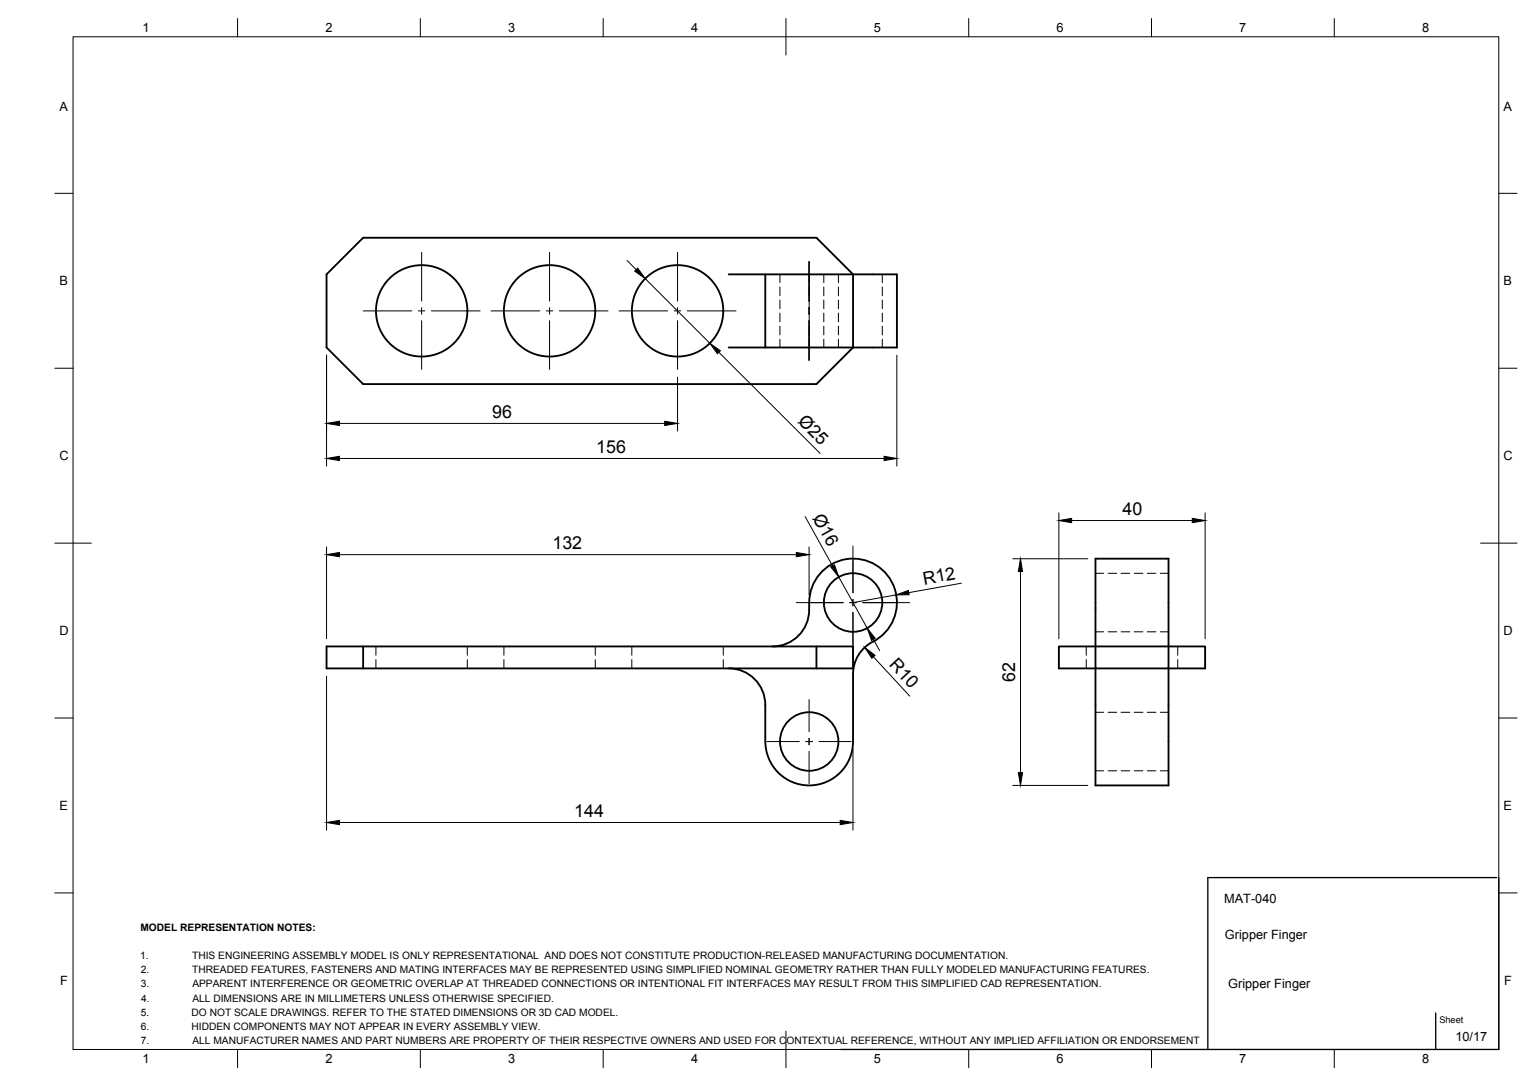
ISO-10303-21;
HEADER;
/* Generated by software containing ST-Developer
 * from STEP Tools, Inc. (www.steptools.com) 
 */

FILE_DESCRIPTION(
/* description */ ('STEP AP214'),
/* implementation_level */ '2;1');

FILE_NAME(
/* name */ 'Gripper Finger.step',
/* time_stamp */ '2026-11-14T21:53:28-08:00',
/* author */ (''),
/* organization */ (''),
/* preprocessor_version */ 'ST-DEVELOPER v20.2',
/* originating_system */ 'Autodesk Translation Framework v15.17.0.0',
/* authorisation */ '');

FILE_SCHEMA (('AUTOMOTIVE_DESIGN { 1 0 10303 214 3 1 1 }'));
ENDSEC;

DATA;
#10=MECHANICAL_DESIGN_GEOMETRIC_PRESENTATION_REPRESENTATION('',(#330),#20176);
#298=SHAPE_REPRESENTATION_RELATIONSHIP('SRR','None',#20261,#310);
#310=ADVANCED_BREP_SHAPE_REPRESENTATION('',(#357),#20167);
#330=STYLED_ITEM('',(#20337),#357);
#357=MANIFOLD_SOLID_BREP('Body1',#10948);
#536=FACE_BOUND('',#2109,.T.);
#537=FACE_BOUND('',#2110,.T.);
#538=FACE_BOUND('',#2111,.T.);
#539=FACE_BOUND('',#2117,.T.);
#540=FACE_BOUND('',#2118,.T.);
#541=FACE_BOUND('',#2119,.T.);
#542=FACE_BOUND('',#2125,.T.);
#543=FACE_BOUND('',#2126,.T.);
#544=FACE_BOUND('',#2128,.T.);
#545=FACE_BOUND('',#2129,.T.);
#826=PLANE('',#11930);
#827=PLANE('',#11931);
#828=PLANE('',#11932);
#829=PLANE('',#11933);
#830=PLANE('',#11934);
#831=PLANE('',#11935);
#832=PLANE('',#11936);
#833=PLANE('',#11940);
#834=PLANE('',#11941);
#835=PLANE('',#11942);
#836=PLANE('',#11946);
#837=PLANE('',#11951);
#838=PLANE('',#11952);
#839=PLANE('',#11953);
#1354=FACE_OUTER_BOUND('',#2102,.T.);
#1355=FACE_OUTER_BOUND('',#2103,.T.);
#1356=FACE_OUTER_BOUND('',#2104,.T.);
#1357=FACE_OUTER_BOUND('',#2105,.T.);
#1358=FACE_OUTER_BOUND('',#2106,.T.);
#1359=FACE_OUTER_BOUND('',#2107,.T.);
#1360=FACE_OUTER_BOUND('',#2108,.T.);
#1361=FACE_OUTER_BOUND('',#2112,.T.);
#1362=FACE_OUTER_BOUND('',#2113,.T.);
#1363=FACE_OUTER_BOUND('',#2114,.T.);
#1364=FACE_OUTER_BOUND('',#2115,.T.);
#1365=FACE_OUTER_BOUND('',#2116,.T.);
#1366=FACE_OUTER_BOUND('',#2120,.T.);
#1367=FACE_OUTER_BOUND('',#2121,.T.);
#1368=FACE_OUTER_BOUND('',#2122,.T.);
#1369=FACE_OUTER_BOUND('',#2123,.T.);
#1370=FACE_OUTER_BOUND('',#2124,.T.);
#1371=FACE_OUTER_BOUND('',#2127,.T.);
#1372=FACE_OUTER_BOUND('',#2130,.T.);
#1373=FACE_OUTER_BOUND('',#2131,.T.);
#1374=FACE_OUTER_BOUND('',#2132,.T.);
#1375=FACE_OUTER_BOUND('',#2133,.T.);
#1376=FACE_OUTER_BOUND('',#2134,.T.);
#1377=FACE_OUTER_BOUND('',#2135,.T.);
#2102=EDGE_LOOP('',(#9561,#9562,#9563,#9564));
#2103=EDGE_LOOP('',(#9565,#9566,#9567,#9568));
#2104=EDGE_LOOP('',(#9569,#9570,#9571,#9572));
#2105=EDGE_LOOP('',(#9573,#9574,#9575,#9576));
#2106=EDGE_LOOP('',(#9577,#9578,#9579,#9580));
#2107=EDGE_LOOP('',(#9581,#9582,#9583,#9584));
#2108=EDGE_LOOP('',(#9585,#9586,#9587,#9588,#9589,#9590,#9591,#9592,#9593,
#9594));
#2109=EDGE_LOOP('',(#9595));
#2110=EDGE_LOOP('',(#9596));
#2111=EDGE_LOOP('',(#9597));
#2112=EDGE_LOOP('',(#9598,#9599,#9600,#9601));
#2113=EDGE_LOOP('',(#9602,#9603,#9604,#9605));
#2114=EDGE_LOOP('',(#9606,#9607,#9608,#9609));
#2115=EDGE_LOOP('',(#9610,#9611,#9612,#9613));
#2116=EDGE_LOOP('',(#9614,#9615,#9616,#9617,#9618,#9619,#9620,#9621,#9622,
#9623));
#2117=EDGE_LOOP('',(#9624));
#2118=EDGE_LOOP('',(#9625));
#2119=EDGE_LOOP('',(#9626));
#2120=EDGE_LOOP('',(#9627,#9628,#9629,#9630));
#2121=EDGE_LOOP('',(#9631,#9632,#9633,#9634));
#2122=EDGE_LOOP('',(#9635,#9636,#9637,#9638));
#2123=EDGE_LOOP('',(#9639,#9640,#9641,#9642));
#2124=EDGE_LOOP('',(#9643,#9644,#9645,#9646,#9647,#9648,#9649,#9650,#9651,
#9652,#9653));
#2125=EDGE_LOOP('',(#9654));
#2126=EDGE_LOOP('',(#9655));
#2127=EDGE_LOOP('',(#9656,#9657,#9658,#9659,#9660,#9661,#9662,#9663,#9664,
#9665,#9666));
#2128=EDGE_LOOP('',(#9667));
#2129=EDGE_LOOP('',(#9668));
#2130=EDGE_LOOP('',(#9669,#9670,#9671,#9672));
#2131=EDGE_LOOP('',(#9673,#9674,#9675,#9676));
#2132=EDGE_LOOP('',(#9677,#9678,#9679,#9680));
#2133=EDGE_LOOP('',(#9681,#9682,#9683,#9684));
#2134=EDGE_LOOP('',(#9685,#9686,#9687,#9688));
#2135=EDGE_LOOP('',(#9689,#9690,#9691,#9692));
#3088=LINE('',#19463,#4076);
#3089=LINE('',#19469,#4077);
#3090=LINE('',#19475,#4078);
#3091=LINE('',#19482,#4079);
#3092=LINE('',#19485,#4080);
#3093=LINE('',#19490,#4081);
#3094=LINE('',#19496,#4082);
#3095=LINE('',#19501,#4083);
#3096=LINE('',#19503,#4084);
#3097=LINE('',#19505,#4085);
#3098=LINE('',#19507,#4086);
#3099=LINE('',#19509,#4087);
#3100=LINE('',#19511,#4088);
#3101=LINE('',#19513,#4089);
#3102=LINE('',#19515,#4090);
#3103=LINE('',#19517,#4091);
#3104=LINE('',#19518,#4092);
#3105=LINE('',#19521,#4093);
#3106=LINE('',#19523,#4094);
#3107=LINE('',#19524,#4095);
#3108=LINE('',#19527,#4096);
#3109=LINE('',#19529,#4097);
#3110=LINE('',#19530,#4098);
#3111=LINE('',#19534,#4099);
#3112=LINE('',#19536,#4100);
#3113=LINE('',#19538,#4101);
#3114=LINE('',#19539,#4102);
#3115=LINE('',#19542,#4103);
#3116=LINE('',#19544,#4104);
#3117=LINE('',#19545,#4105);
#3118=LINE('',#19548,#4106);
#3119=LINE('',#19550,#4107);
#3120=LINE('',#19552,#4108);
#3121=LINE('',#19554,#4109);
#3122=LINE('',#19555,#4110);
#3123=LINE('',#19556,#4111);
#3124=LINE('',#19557,#4112);
#3125=LINE('',#19561,#4113);
#3126=LINE('',#19563,#4114);
#3127=LINE('',#19565,#4115);
#3128=LINE('',#19566,#4116);
#3129=LINE('',#19575,#4117);
#3130=LINE('',#19577,#4118);
#3131=LINE('',#19581,#4119);
#3132=LINE('',#19584,#4120);
#3133=LINE('',#19590,#4121);
#4076=VECTOR('',#14642,12.5);
#4077=VECTOR('',#14649,12.5);
#4078=VECTOR('',#14656,12.5);
#4079=VECTOR('',#14663,1000.);
#4080=VECTOR('',#14666,1000.);
#4081=VECTOR('',#14671,8.);
#4082=VECTOR('',#14678,8.);
#4083=VECTOR('',#14683,1000.);
#4084=VECTOR('',#14684,1000.);
#4085=VECTOR('',#14685,1000.);
#4086=VECTOR('',#14686,1000.);
#4087=VECTOR('',#14687,1000.);
#4088=VECTOR('',#14688,1000.);
#4089=VECTOR('',#14689,1000.);
#4090=VECTOR('',#14690,1000.);
#4091=VECTOR('',#14691,1000.);
#4092=VECTOR('',#14692,1000.);
#4093=VECTOR('',#14695,1000.);
#4094=VECTOR('',#14696,1000.);
#4095=VECTOR('',#14697,1000.);
#4096=VECTOR('',#14700,1000.);
#4097=VECTOR('',#14701,1000.);
#4098=VECTOR('',#14702,1000.);
#4099=VECTOR('',#14705,1000.);
#4100=VECTOR('',#14706,1000.);
#4101=VECTOR('',#14707,1000.);
#4102=VECTOR('',#14708,1000.);
#4103=VECTOR('',#14711,1000.);
#4104=VECTOR('',#14712,1000.);
#4105=VECTOR('',#14713,1000.);
#4106=VECTOR('',#14716,1000.);
#4107=VECTOR('',#14717,1000.);
#4108=VECTOR('',#14718,1000.);
#4109=VECTOR('',#14719,1000.);
#4110=VECTOR('',#14720,1000.);
#4111=VECTOR('',#14721,1000.);
#4112=VECTOR('',#14722,1000.);
#4113=VECTOR('',#14725,1000.);
#4114=VECTOR('',#14726,1000.);
#4115=VECTOR('',#14727,1000.);
#4116=VECTOR('',#14728,1000.);
#4117=VECTOR('',#14743,1000.);
#4118=VECTOR('',#14746,1000.);
#4119=VECTOR('',#14751,1000.);
#4120=VECTOR('',#14756,1000.);
#4121=VECTOR('',#14767,1000.);
#4615=CIRCLE('',#11913,12.5);
#4616=CIRCLE('',#11914,12.5);
#4617=CIRCLE('',#11916,12.5);
#4618=CIRCLE('',#11917,12.5);
#4619=CIRCLE('',#11919,12.5);
#4620=CIRCLE('',#11920,12.5);
#4621=CIRCLE('',#11922,12.);
#4622=CIRCLE('',#11923,12.);
#4623=CIRCLE('',#11925,8.);
#4624=CIRCLE('',#11926,8.);
#4625=CIRCLE('',#11928,8.);
#4626=CIRCLE('',#11929,8.);
#4627=CIRCLE('',#11938,12.);
#4628=CIRCLE('',#11939,12.);
#4629=CIRCLE('',#11943,10.);
#4630=CIRCLE('',#11944,10.);
#4631=CIRCLE('',#11945,10.);
#4632=CIRCLE('',#11947,10.);
#4633=CIRCLE('',#11948,10.);
#4634=CIRCLE('',#11949,10.);
#5490=VERTEX_POINT('',#19460);
#5491=VERTEX_POINT('',#19462);
#5492=VERTEX_POINT('',#19466);
#5493=VERTEX_POINT('',#19468);
#5494=VERTEX_POINT('',#19472);
#5495=VERTEX_POINT('',#19474);
#5496=VERTEX_POINT('',#19478);
#5497=VERTEX_POINT('',#19479);
#5498=VERTEX_POINT('',#19481);
#5499=VERTEX_POINT('',#19483);
#5500=VERTEX_POINT('',#19487);
#5501=VERTEX_POINT('',#19489);
#5502=VERTEX_POINT('',#19493);
#5503=VERTEX_POINT('',#19495);
#5504=VERTEX_POINT('',#19499);
#5505=VERTEX_POINT('',#19500);
#5506=VERTEX_POINT('',#19502);
#5507=VERTEX_POINT('',#19504);
#5508=VERTEX_POINT('',#19506);
#5509=VERTEX_POINT('',#19508);
#5510=VERTEX_POINT('',#19510);
#5511=VERTEX_POINT('',#19512);
#5512=VERTEX_POINT('',#19514);
#5513=VERTEX_POINT('',#19516);
#5514=VERTEX_POINT('',#19520);
#5515=VERTEX_POINT('',#19522);
#5516=VERTEX_POINT('',#19526);
#5517=VERTEX_POINT('',#19528);
#5518=VERTEX_POINT('',#19532);
#5519=VERTEX_POINT('',#19533);
#5520=VERTEX_POINT('',#19535);
#5521=VERTEX_POINT('',#19537);
#5522=VERTEX_POINT('',#19541);
#5523=VERTEX_POINT('',#19543);
#5524=VERTEX_POINT('',#19547);
#5525=VERTEX_POINT('',#19549);
#5526=VERTEX_POINT('',#19551);
#5527=VERTEX_POINT('',#19553);
#5528=VERTEX_POINT('',#19559);
#5529=VERTEX_POINT('',#19560);
#5530=VERTEX_POINT('',#19562);
#5531=VERTEX_POINT('',#19564);
#5532=VERTEX_POINT('',#19574);
#5533=VERTEX_POINT('',#19580);
#6891=EDGE_CURVE('',#5490,#5490,#4615,.T.);
#6892=EDGE_CURVE('',#5490,#5491,#3088,.T.);
#6893=EDGE_CURVE('',#5491,#5491,#4616,.T.);
#6894=EDGE_CURVE('',#5492,#5492,#4617,.T.);
#6895=EDGE_CURVE('',#5492,#5493,#3089,.T.);
#6896=EDGE_CURVE('',#5493,#5493,#4618,.T.);
#6897=EDGE_CURVE('',#5494,#5494,#4619,.T.);
#6898=EDGE_CURVE('',#5494,#5495,#3090,.T.);
#6899=EDGE_CURVE('',#5495,#5495,#4620,.T.);
#6900=EDGE_CURVE('',#5496,#5497,#4621,.T.);
#6901=EDGE_CURVE('',#5497,#5498,#3091,.T.);
#6902=EDGE_CURVE('',#5498,#5499,#4622,.T.);
#6903=EDGE_CURVE('',#5499,#5496,#3092,.T.);
#6904=EDGE_CURVE('',#5500,#5500,#4623,.T.);
#6905=EDGE_CURVE('',#5500,#5501,#3093,.T.);
#6906=EDGE_CURVE('',#5501,#5501,#4624,.T.);
#6907=EDGE_CURVE('',#5502,#5502,#4625,.T.);
#6908=EDGE_CURVE('',#5502,#5503,#3094,.T.);
#6909=EDGE_CURVE('',#5503,#5503,#4626,.T.);
#6910=EDGE_CURVE('',#5504,#5505,#3095,.T.);
#6911=EDGE_CURVE('',#5505,#5506,#3096,.T.);
#6912=EDGE_CURVE('',#5507,#5506,#3097,.T.);
#6913=EDGE_CURVE('',#5508,#5507,#3098,.T.);
#6914=EDGE_CURVE('',#5508,#5509,#3099,.T.);
#6915=EDGE_CURVE('',#5509,#5510,#3100,.T.);
#6916=EDGE_CURVE('',#5511,#5510,#3101,.T.);
#6917=EDGE_CURVE('',#5511,#5512,#3102,.T.);
#6918=EDGE_CURVE('',#5513,#5512,#3103,.T.);
#6919=EDGE_CURVE('',#5504,#5513,#3104,.T.);
#6920=EDGE_CURVE('',#5513,#5514,#3105,.T.);
#6921=EDGE_CURVE('',#5512,#5515,#3106,.T.);
#6922=EDGE_CURVE('',#5515,#5514,#3107,.T.);
#6923=EDGE_CURVE('',#5508,#5516,#3108,.T.);
#6924=EDGE_CURVE('',#5517,#5516,#3109,.T.);
#6925=EDGE_CURVE('',#5517,#5509,#3110,.T.);
#6926=EDGE_CURVE('',#5518,#5519,#3111,.T.);
#6927=EDGE_CURVE('',#5518,#5520,#3112,.T.);
#6928=EDGE_CURVE('',#5521,#5520,#3113,.T.);
#6929=EDGE_CURVE('',#5521,#5519,#3114,.T.);
#6930=EDGE_CURVE('',#5510,#5522,#3115,.T.);
#6931=EDGE_CURVE('',#5523,#5522,#3116,.T.);
#6932=EDGE_CURVE('',#5523,#5511,#3117,.T.);
#6933=EDGE_CURVE('',#5524,#5516,#3118,.T.);
#6934=EDGE_CURVE('',#5524,#5525,#3119,.T.);
#6935=EDGE_CURVE('',#5525,#5526,#3120,.T.);
#6936=EDGE_CURVE('',#5527,#5526,#3121,.T.);
#6937=EDGE_CURVE('',#5514,#5527,#3122,.T.);
#6938=EDGE_CURVE('',#5515,#5523,#3123,.T.);
#6939=EDGE_CURVE('',#5522,#5517,#3124,.T.);
#6940=EDGE_CURVE('',#5528,#5529,#3125,.T.);
#6941=EDGE_CURVE('',#5528,#5530,#3126,.T.);
#6942=EDGE_CURVE('',#5531,#5530,#3127,.T.);
#6943=EDGE_CURVE('',#5529,#5531,#3128,.T.);
#6944=EDGE_CURVE('',#5519,#5531,#4627,.T.);
#6945=EDGE_CURVE('',#5529,#5521,#4628,.T.);
#6946=EDGE_CURVE('',#5520,#5499,#4629,.T.);
#6947=EDGE_CURVE('',#5532,#5498,#3129,.T.);
#6948=EDGE_CURVE('',#5532,#5505,#4630,.T.);
#6949=EDGE_CURVE('',#5504,#5527,#3130,.T.);
#6950=EDGE_CURVE('',#5526,#5528,#4631,.T.);
#6951=EDGE_CURVE('',#5497,#5533,#3131,.T.);
#6952=EDGE_CURVE('',#5496,#5518,#4632,.T.);
#6953=EDGE_CURVE('',#5530,#5525,#4633,.T.);
#6954=EDGE_CURVE('',#5507,#5524,#3132,.T.);
#6955=EDGE_CURVE('',#5506,#5533,#4634,.T.);
#6956=EDGE_CURVE('',#5533,#5532,#3133,.T.);
#9561=ORIENTED_EDGE('',*,*,#6891,.T.);
#9562=ORIENTED_EDGE('',*,*,#6892,.T.);
#9563=ORIENTED_EDGE('',*,*,#6893,.T.);
#9564=ORIENTED_EDGE('',*,*,#6892,.F.);
#9565=ORIENTED_EDGE('',*,*,#6894,.T.);
#9566=ORIENTED_EDGE('',*,*,#6895,.T.);
#9567=ORIENTED_EDGE('',*,*,#6896,.T.);
#9568=ORIENTED_EDGE('',*,*,#6895,.F.);
#9569=ORIENTED_EDGE('',*,*,#6897,.T.);
#9570=ORIENTED_EDGE('',*,*,#6898,.T.);
#9571=ORIENTED_EDGE('',*,*,#6899,.T.);
#9572=ORIENTED_EDGE('',*,*,#6898,.F.);
#9573=ORIENTED_EDGE('',*,*,#6900,.T.);
#9574=ORIENTED_EDGE('',*,*,#6901,.T.);
#9575=ORIENTED_EDGE('',*,*,#6902,.T.);
#9576=ORIENTED_EDGE('',*,*,#6903,.T.);
#9577=ORIENTED_EDGE('',*,*,#6904,.F.);
#9578=ORIENTED_EDGE('',*,*,#6905,.T.);
#9579=ORIENTED_EDGE('',*,*,#6906,.F.);
#9580=ORIENTED_EDGE('',*,*,#6905,.F.);
#9581=ORIENTED_EDGE('',*,*,#6907,.T.);
#9582=ORIENTED_EDGE('',*,*,#6908,.T.);
#9583=ORIENTED_EDGE('',*,*,#6909,.T.);
#9584=ORIENTED_EDGE('',*,*,#6908,.F.);
#9585=ORIENTED_EDGE('',*,*,#6910,.T.);
#9586=ORIENTED_EDGE('',*,*,#6911,.T.);
#9587=ORIENTED_EDGE('',*,*,#6912,.F.);
#9588=ORIENTED_EDGE('',*,*,#6913,.F.);
#9589=ORIENTED_EDGE('',*,*,#6914,.T.);
#9590=ORIENTED_EDGE('',*,*,#6915,.T.);
#9591=ORIENTED_EDGE('',*,*,#6916,.F.);
#9592=ORIENTED_EDGE('',*,*,#6917,.T.);
#9593=ORIENTED_EDGE('',*,*,#6918,.F.);
#9594=ORIENTED_EDGE('',*,*,#6919,.F.);
#9595=ORIENTED_EDGE('',*,*,#6893,.F.);
#9596=ORIENTED_EDGE('',*,*,#6896,.F.);
#9597=ORIENTED_EDGE('',*,*,#6899,.F.);
#9598=ORIENTED_EDGE('',*,*,#6920,.F.);
#9599=ORIENTED_EDGE('',*,*,#6918,.T.);
#9600=ORIENTED_EDGE('',*,*,#6921,.T.);
#9601=ORIENTED_EDGE('',*,*,#6922,.T.);
#9602=ORIENTED_EDGE('',*,*,#6914,.F.);
#9603=ORIENTED_EDGE('',*,*,#6923,.T.);
#9604=ORIENTED_EDGE('',*,*,#6924,.F.);
#9605=ORIENTED_EDGE('',*,*,#6925,.T.);
#9606=ORIENTED_EDGE('',*,*,#6926,.F.);
#9607=ORIENTED_EDGE('',*,*,#6927,.T.);
#9608=ORIENTED_EDGE('',*,*,#6928,.F.);
#9609=ORIENTED_EDGE('',*,*,#6929,.T.);
#9610=ORIENTED_EDGE('',*,*,#6916,.T.);
#9611=ORIENTED_EDGE('',*,*,#6930,.T.);
#9612=ORIENTED_EDGE('',*,*,#6931,.F.);
#9613=ORIENTED_EDGE('',*,*,#6932,.T.);
#9614=ORIENTED_EDGE('',*,*,#6924,.T.);
#9615=ORIENTED_EDGE('',*,*,#6933,.F.);
#9616=ORIENTED_EDGE('',*,*,#6934,.T.);
#9617=ORIENTED_EDGE('',*,*,#6935,.T.);
#9618=ORIENTED_EDGE('',*,*,#6936,.F.);
#9619=ORIENTED_EDGE('',*,*,#6937,.F.);
#9620=ORIENTED_EDGE('',*,*,#6922,.F.);
#9621=ORIENTED_EDGE('',*,*,#6938,.T.);
#9622=ORIENTED_EDGE('',*,*,#6931,.T.);
#9623=ORIENTED_EDGE('',*,*,#6939,.T.);
#9624=ORIENTED_EDGE('',*,*,#6891,.F.);
#9625=ORIENTED_EDGE('',*,*,#6894,.F.);
#9626=ORIENTED_EDGE('',*,*,#6897,.F.);
#9627=ORIENTED_EDGE('',*,*,#6940,.F.);
#9628=ORIENTED_EDGE('',*,*,#6941,.T.);
#9629=ORIENTED_EDGE('',*,*,#6942,.F.);
#9630=ORIENTED_EDGE('',*,*,#6943,.F.);
#9631=ORIENTED_EDGE('',*,*,#6943,.T.);
#9632=ORIENTED_EDGE('',*,*,#6944,.F.);
#9633=ORIENTED_EDGE('',*,*,#6929,.F.);
#9634=ORIENTED_EDGE('',*,*,#6945,.F.);
#9635=ORIENTED_EDGE('',*,*,#6915,.F.);
#9636=ORIENTED_EDGE('',*,*,#6925,.F.);
#9637=ORIENTED_EDGE('',*,*,#6939,.F.);
#9638=ORIENTED_EDGE('',*,*,#6930,.F.);
#9639=ORIENTED_EDGE('',*,*,#6917,.F.);
#9640=ORIENTED_EDGE('',*,*,#6932,.F.);
#9641=ORIENTED_EDGE('',*,*,#6938,.F.);
#9642=ORIENTED_EDGE('',*,*,#6921,.F.);
#9643=ORIENTED_EDGE('',*,*,#6928,.T.);
#9644=ORIENTED_EDGE('',*,*,#6946,.T.);
#9645=ORIENTED_EDGE('',*,*,#6902,.F.);
#9646=ORIENTED_EDGE('',*,*,#6947,.F.);
#9647=ORIENTED_EDGE('',*,*,#6948,.T.);
#9648=ORIENTED_EDGE('',*,*,#6910,.F.);
#9649=ORIENTED_EDGE('',*,*,#6949,.T.);
#9650=ORIENTED_EDGE('',*,*,#6936,.T.);
#9651=ORIENTED_EDGE('',*,*,#6950,.T.);
#9652=ORIENTED_EDGE('',*,*,#6940,.T.);
#9653=ORIENTED_EDGE('',*,*,#6945,.T.);
#9654=ORIENTED_EDGE('',*,*,#6906,.T.);
#9655=ORIENTED_EDGE('',*,*,#6907,.F.);
#9656=ORIENTED_EDGE('',*,*,#6951,.F.);
#9657=ORIENTED_EDGE('',*,*,#6900,.F.);
#9658=ORIENTED_EDGE('',*,*,#6952,.T.);
#9659=ORIENTED_EDGE('',*,*,#6926,.T.);
#9660=ORIENTED_EDGE('',*,*,#6944,.T.);
#9661=ORIENTED_EDGE('',*,*,#6942,.T.);
#9662=ORIENTED_EDGE('',*,*,#6953,.T.);
#9663=ORIENTED_EDGE('',*,*,#6934,.F.);
#9664=ORIENTED_EDGE('',*,*,#6954,.F.);
#9665=ORIENTED_EDGE('',*,*,#6912,.T.);
#9666=ORIENTED_EDGE('',*,*,#6955,.T.);
#9667=ORIENTED_EDGE('',*,*,#6904,.T.);
#9668=ORIENTED_EDGE('',*,*,#6909,.F.);
#9669=ORIENTED_EDGE('',*,*,#6950,.F.);
#9670=ORIENTED_EDGE('',*,*,#6935,.F.);
#9671=ORIENTED_EDGE('',*,*,#6953,.F.);
#9672=ORIENTED_EDGE('',*,*,#6941,.F.);
#9673=ORIENTED_EDGE('',*,*,#6919,.T.);
#9674=ORIENTED_EDGE('',*,*,#6920,.T.);
#9675=ORIENTED_EDGE('',*,*,#6937,.T.);
#9676=ORIENTED_EDGE('',*,*,#6949,.F.);
#9677=ORIENTED_EDGE('',*,*,#6913,.T.);
#9678=ORIENTED_EDGE('',*,*,#6954,.T.);
#9679=ORIENTED_EDGE('',*,*,#6933,.T.);
#9680=ORIENTED_EDGE('',*,*,#6923,.F.);
#9681=ORIENTED_EDGE('',*,*,#6951,.T.);
#9682=ORIENTED_EDGE('',*,*,#6956,.T.);
#9683=ORIENTED_EDGE('',*,*,#6947,.T.);
#9684=ORIENTED_EDGE('',*,*,#6901,.F.);
#9685=ORIENTED_EDGE('',*,*,#6955,.F.);
#9686=ORIENTED_EDGE('',*,*,#6911,.F.);
#9687=ORIENTED_EDGE('',*,*,#6948,.F.);
#9688=ORIENTED_EDGE('',*,*,#6956,.F.);
#9689=ORIENTED_EDGE('',*,*,#6946,.F.);
#9690=ORIENTED_EDGE('',*,*,#6927,.F.);
#9691=ORIENTED_EDGE('',*,*,#6952,.F.);
#9692=ORIENTED_EDGE('',*,*,#6903,.F.);
#10311=CYLINDRICAL_SURFACE('',#11912,12.5);
#10312=CYLINDRICAL_SURFACE('',#11915,12.5);
#10313=CYLINDRICAL_SURFACE('',#11918,12.5);
#10314=CYLINDRICAL_SURFACE('',#11921,12.);
#10315=CYLINDRICAL_SURFACE('',#11924,8.);
#10316=CYLINDRICAL_SURFACE('',#11927,8.);
#10317=CYLINDRICAL_SURFACE('',#11937,12.);
#10318=CYLINDRICAL_SURFACE('',#11950,10.);
#10319=CYLINDRICAL_SURFACE('',#11954,10.);
#10320=CYLINDRICAL_SURFACE('',#11955,10.);
#10806=ADVANCED_FACE('',(#1354),#10311,.F.);
#10807=ADVANCED_FACE('',(#1355),#10312,.F.);
#10808=ADVANCED_FACE('',(#1356),#10313,.F.);
#10809=ADVANCED_FACE('',(#1357),#10314,.T.);
#10810=ADVANCED_FACE('',(#1358),#10315,.F.);
#10811=ADVANCED_FACE('',(#1359),#10316,.F.);
#10812=ADVANCED_FACE('',(#1360,#536,#537,#538),#826,.F.);
#10813=ADVANCED_FACE('',(#1361),#827,.T.);
#10814=ADVANCED_FACE('',(#1362),#828,.F.);
#10815=ADVANCED_FACE('',(#1363),#829,.F.);
#10816=ADVANCED_FACE('',(#1364),#830,.F.);
#10817=ADVANCED_FACE('',(#1365,#539,#540,#541),#831,.F.);
#10818=ADVANCED_FACE('',(#1366),#832,.F.);
#10819=ADVANCED_FACE('',(#1367),#10317,.T.);
#10820=ADVANCED_FACE('',(#1368),#833,.F.);
#10821=ADVANCED_FACE('',(#1369),#834,.T.);
#10822=ADVANCED_FACE('',(#1370,#542,#543),#835,.F.);
#10823=ADVANCED_FACE('',(#1371,#544,#545),#836,.F.);
#10824=ADVANCED_FACE('',(#1372),#10318,.F.);
#10825=ADVANCED_FACE('',(#1373),#837,.F.);
#10826=ADVANCED_FACE('',(#1374),#838,.F.);
#10827=ADVANCED_FACE('',(#1375),#839,.F.);
#10828=ADVANCED_FACE('',(#1376),#10319,.F.);
#10829=ADVANCED_FACE('',(#1377),#10320,.F.);
#10948=CLOSED_SHELL('',(#10806,#10807,#10808,#10809,#10810,#10811,#10812,
#10813,#10814,#10815,#10816,#10817,#10818,#10819,#10820,#10821,#10822,#10823,
#10824,#10825,#10826,#10827,#10828,#10829));
#11911=AXIS2_PLACEMENT_3D('',#19458,#14636,#14637);
#11912=AXIS2_PLACEMENT_3D('',#19459,#14638,#14639);
#11913=AXIS2_PLACEMENT_3D('',#19461,#14640,#14641);
#11914=AXIS2_PLACEMENT_3D('',#19464,#14643,#14644);
#11915=AXIS2_PLACEMENT_3D('',#19465,#14645,#14646);
#11916=AXIS2_PLACEMENT_3D('',#19467,#14647,#14648);
#11917=AXIS2_PLACEMENT_3D('',#19470,#14650,#14651);
#11918=AXIS2_PLACEMENT_3D('',#19471,#14652,#14653);
#11919=AXIS2_PLACEMENT_3D('',#19473,#14654,#14655);
#11920=AXIS2_PLACEMENT_3D('',#19476,#14657,#14658);
#11921=AXIS2_PLACEMENT_3D('',#19477,#14659,#14660);
#11922=AXIS2_PLACEMENT_3D('',#19480,#14661,#14662);
#11923=AXIS2_PLACEMENT_3D('',#19484,#14664,#14665);
#11924=AXIS2_PLACEMENT_3D('',#19486,#14667,#14668);
#11925=AXIS2_PLACEMENT_3D('',#19488,#14669,#14670);
#11926=AXIS2_PLACEMENT_3D('',#19491,#14672,#14673);
#11927=AXIS2_PLACEMENT_3D('',#19492,#14674,#14675);
#11928=AXIS2_PLACEMENT_3D('',#19494,#14676,#14677);
#11929=AXIS2_PLACEMENT_3D('',#19497,#14679,#14680);
#11930=AXIS2_PLACEMENT_3D('',#19498,#14681,#14682);
#11931=AXIS2_PLACEMENT_3D('',#19519,#14693,#14694);
#11932=AXIS2_PLACEMENT_3D('',#19525,#14698,#14699);
#11933=AXIS2_PLACEMENT_3D('',#19531,#14703,#14704);
#11934=AXIS2_PLACEMENT_3D('',#19540,#14709,#14710);
#11935=AXIS2_PLACEMENT_3D('',#19546,#14714,#14715);
#11936=AXIS2_PLACEMENT_3D('',#19558,#14723,#14724);
#11937=AXIS2_PLACEMENT_3D('',#19567,#14729,#14730);
#11938=AXIS2_PLACEMENT_3D('',#19568,#14731,#14732);
#11939=AXIS2_PLACEMENT_3D('',#19569,#14733,#14734);
#11940=AXIS2_PLACEMENT_3D('',#19570,#14735,#14736);
#11941=AXIS2_PLACEMENT_3D('',#19571,#14737,#14738);
#11942=AXIS2_PLACEMENT_3D('',#19572,#14739,#14740);
#11943=AXIS2_PLACEMENT_3D('',#19573,#14741,#14742);
#11944=AXIS2_PLACEMENT_3D('',#19576,#14744,#14745);
#11945=AXIS2_PLACEMENT_3D('',#19578,#14747,#14748);
#11946=AXIS2_PLACEMENT_3D('',#19579,#14749,#14750);
#11947=AXIS2_PLACEMENT_3D('',#19582,#14752,#14753);
#11948=AXIS2_PLACEMENT_3D('',#19583,#14754,#14755);
#11949=AXIS2_PLACEMENT_3D('',#19585,#14757,#14758);
#11950=AXIS2_PLACEMENT_3D('',#19586,#14759,#14760);
#11951=AXIS2_PLACEMENT_3D('',#19587,#14761,#14762);
#11952=AXIS2_PLACEMENT_3D('',#19588,#14763,#14764);
#11953=AXIS2_PLACEMENT_3D('',#19589,#14765,#14766);
#11954=AXIS2_PLACEMENT_3D('',#19591,#14768,#14769);
#11955=AXIS2_PLACEMENT_3D('',#19592,#14770,#14771);
#14636=DIRECTION('axis',(0.,0.,1.));
#14637=DIRECTION('refdir',(1.,0.,0.));
#14638=DIRECTION('center_axis',(1.,0.,0.));
#14639=DIRECTION('ref_axis',(0.,0.,-1.));
#14640=DIRECTION('center_axis',(-1.,0.,0.));
#14641=DIRECTION('ref_axis',(0.,0.,-1.));
#14642=DIRECTION('',(1.,0.,0.));
#14643=DIRECTION('center_axis',(1.,0.,0.));
#14644=DIRECTION('ref_axis',(0.,0.,1.));
#14645=DIRECTION('center_axis',(1.,0.,0.));
#14646=DIRECTION('ref_axis',(0.,0.,-1.));
#14647=DIRECTION('center_axis',(-1.,0.,0.));
#14648=DIRECTION('ref_axis',(0.,0.,-1.));
#14649=DIRECTION('',(1.,0.,0.));
#14650=DIRECTION('center_axis',(1.,0.,0.));
#14651=DIRECTION('ref_axis',(0.,0.,-1.));
#14652=DIRECTION('center_axis',(1.,0.,0.));
#14653=DIRECTION('ref_axis',(0.,0.,-1.));
#14654=DIRECTION('center_axis',(-1.,0.,0.));
#14655=DIRECTION('ref_axis',(0.,0.,-1.));
#14656=DIRECTION('',(1.,0.,0.));
#14657=DIRECTION('center_axis',(1.,0.,0.));
#14658=DIRECTION('ref_axis',(0.,0.,-1.));
#14659=DIRECTION('center_axis',(0.,1.,0.));
#14660=DIRECTION('ref_axis',(0.,0.,1.));
#14661=DIRECTION('center_axis',(3.46944695195361E-16,1.,0.));
#14662=DIRECTION('ref_axis',(-1.,3.46944695195361E-16,0.));
#14663=DIRECTION('',(-1.73472347597681E-16,1.,0.));
#14664=DIRECTION('center_axis',(1.73472347597681E-16,-1.,0.));
#14665=DIRECTION('ref_axis',(1.,1.73472347597681E-16,0.));
#14666=DIRECTION('',(0.,-1.,0.));
#14667=DIRECTION('center_axis',(0.,1.,0.));
#14668=DIRECTION('ref_axis',(0.,0.,1.));
#14669=DIRECTION('center_axis',(3.46944695195361E-16,1.,0.));
#14670=DIRECTION('ref_axis',(-1.,3.46944695195361E-16,0.));
#14671=DIRECTION('',(0.,1.,0.));
#14672=DIRECTION('center_axis',(1.73472347597681E-16,-1.,0.));
#14673=DIRECTION('ref_axis',(1.,1.73472347597681E-16,0.));
#14674=DIRECTION('center_axis',(0.,-1.,0.));
#14675=DIRECTION('ref_axis',(0.,0.,-1.));
#14676=DIRECTION('center_axis',(0.,1.,0.));
#14677=DIRECTION('ref_axis',(0.,0.,-1.));
#14678=DIRECTION('',(0.,-1.,0.));
#14679=DIRECTION('center_axis',(0.,-1.,0.));
#14680=DIRECTION('ref_axis',(0.,0.,1.));
#14681=DIRECTION('center_axis',(-1.,0.,0.));
#14682=DIRECTION('ref_axis',(0.,0.,1.));
#14683=DIRECTION('',(0.,0.,-1.));
#14684=DIRECTION('',(0.,-1.,5.01544256350842E-32));
#14685=DIRECTION('',(0.,0.,-1.));
#14686=DIRECTION('',(0.,0.707106781186548,0.707106781186548));
#14687=DIRECTION('',(0.,0.,-1.));
#14688=DIRECTION('',(0.,0.707106781186546,-0.707106781186549));
#14689=DIRECTION('',(0.,-1.,0.));
#14690=DIRECTION('',(0.,0.707106781186547,0.707106781186547));
#14691=DIRECTION('',(0.,0.,-1.));
#14692=DIRECTION('',(0.,0.707106781186547,-0.707106781186548));
#14693=DIRECTION('center_axis',(0.,1.,0.));
#14694=DIRECTION('ref_axis',(0.,0.,1.));
#14695=DIRECTION('',(-1.,0.,0.));
#14696=DIRECTION('',(-1.,0.,0.));
#14697=DIRECTION('',(0.,0.,1.));
#14698=DIRECTION('center_axis',(0.,1.,0.));
#14699=DIRECTION('ref_axis',(0.,0.,1.));
#14700=DIRECTION('',(-1.,0.,0.));
#14701=DIRECTION('',(0.,0.,1.));
#14702=DIRECTION('',(1.,0.,0.));
#14703=DIRECTION('center_axis',(-4.00320802148494E-16,0.,-1.));
#14704=DIRECTION('ref_axis',(-1.,0.,4.00320802148494E-16));
#14705=DIRECTION('',(-1.,0.,4.00320802148494E-16));
#14706=DIRECTION('',(0.,1.,0.));
#14707=DIRECTION('',(1.,0.,-4.00320802148494E-16));
#14708=DIRECTION('',(0.,-1.,0.));
#14709=DIRECTION('center_axis',(0.,0.,1.));
#14710=DIRECTION('ref_axis',(1.,0.,0.));
#14711=DIRECTION('',(-1.,0.,0.));
#14712=DIRECTION('',(0.,-1.,0.));
#14713=DIRECTION('',(1.,0.,0.));
#14714=DIRECTION('center_axis',(1.,0.,0.));
#14715=DIRECTION('ref_axis',(0.,0.,-1.));
#14716=DIRECTION('',(0.,-0.707106781186548,-0.707106781186548));
#14717=DIRECTION('',(0.,0.,-1.));
#14718=DIRECTION('',(0.,1.,0.));
#14719=DIRECTION('',(0.,0.,-1.));
#14720=DIRECTION('',(0.,-0.707106781186547,0.707106781186548));
#14721=DIRECTION('',(0.,-0.707106781186547,-0.707106781186547));
#14722=DIRECTION('',(0.,-0.707106781186546,0.707106781186549));
#14723=DIRECTION('center_axis',(0.,0.,1.));
#14724=DIRECTION('ref_axis',(1.,0.,0.));
#14725=DIRECTION('',(-1.,0.,0.));
#14726=DIRECTION('',(0.,-1.,0.));
#14727=DIRECTION('',(1.,0.,0.));
#14728=DIRECTION('',(0.,-1.,0.));
#14729=DIRECTION('center_axis',(0.,-1.,0.));
#14730=DIRECTION('ref_axis',(0.,0.,-1.));
#14731=DIRECTION('center_axis',(0.,-1.,0.));
#14732=DIRECTION('ref_axis',(0.,0.,1.));
#14733=DIRECTION('center_axis',(0.,1.,0.));
#14734=DIRECTION('ref_axis',(0.,0.,-1.));
#14735=DIRECTION('center_axis',(0.,0.707106781186549,0.707106781186546));
#14736=DIRECTION('ref_axis',(-1.,0.,0.));
#14737=DIRECTION('center_axis',(0.,0.707106781186548,-0.707106781186548));
#14738=DIRECTION('ref_axis',(1.,0.,0.));
#14739=DIRECTION('center_axis',(0.,-1.,0.));
#14740=DIRECTION('ref_axis',(0.,0.,-1.));
#14741=DIRECTION('center_axis',(1.73472347597681E-16,-1.,0.));
#14742=DIRECTION('ref_axis',(1.,1.73472347597681E-16,0.));
#14743=DIRECTION('',(1.,2.89120579329468E-16,-2.89120579329468E-16));
#14744=DIRECTION('center_axis',(1.73472347597681E-16,-1.,0.));
#14745=DIRECTION('ref_axis',(1.,1.73472347597681E-16,0.));
#14746=DIRECTION('',(-1.,-1.73472347597681E-16,1.73472347597681E-16));
#14747=DIRECTION('center_axis',(0.,-1.,0.));
#14748=DIRECTION('ref_axis',(0.,0.,-1.));
#14749=DIRECTION('center_axis',(3.46944695195361E-16,1.,0.));
#14750=DIRECTION('ref_axis',(-1.,3.46944695195361E-16,0.));
#14751=DIRECTION('',(-1.,3.46944695195361E-16,2.89120579329468E-16));
#14752=DIRECTION('center_axis',(0.,1.,0.));
#14753=DIRECTION('ref_axis',(0.,0.,1.));
#14754=DIRECTION('center_axis',(0.,1.,0.));
#14755=DIRECTION('ref_axis',(0.,0.,1.));
#14756=DIRECTION('',(-1.,3.46944695195361E-16,3.46944695195361E-16));
#14757=DIRECTION('center_axis',(3.46944695195361E-16,1.,0.));
#14758=DIRECTION('ref_axis',(-1.,3.46944695195361E-16,0.));
#14759=DIRECTION('center_axis',(0.,1.,0.));
#14760=DIRECTION('ref_axis',(0.,0.,1.));
#14761=DIRECTION('center_axis',(0.,-0.707106781186548,-0.707106781186547));
#14762=DIRECTION('ref_axis',(0.,0.707106781186547,-0.707106781186548));
#14763=DIRECTION('center_axis',(0.,0.707106781186547,-0.707106781186548));
#14764=DIRECTION('ref_axis',(0.,0.707106781186548,0.707106781186547));
#14765=DIRECTION('center_axis',(2.89120579329468E-16,5.01544256350842E-32,
1.));
#14766=DIRECTION('ref_axis',(1.,-1.72766579818696E-64,-2.89120579329468E-16));
#14767=DIRECTION('',(0.,1.,-5.01544256350842E-32));
#14768=DIRECTION('center_axis',(0.,-1.,5.01544256350842E-32));
#14769=DIRECTION('ref_axis',(0.,-5.01544256350842E-32,-1.));
#14770=DIRECTION('center_axis',(0.,1.,0.));
#14771=DIRECTION('ref_axis',(0.,0.,1.));
#19458=CARTESIAN_POINT('',(0.,0.,0.));
#19459=CARTESIAN_POINT('Origin',(-38.001,20.,-48.));
#19460=CARTESIAN_POINT('',(-6.,20.,-35.5));
#19461=CARTESIAN_POINT('Origin',(-6.,20.,-48.));
#19462=CARTESIAN_POINT('',(0.,20.,-35.5));
#19463=CARTESIAN_POINT('',(-38.001,20.,-35.5));
#19464=CARTESIAN_POINT('Origin',(0.,20.,-48.));
#19465=CARTESIAN_POINT('Origin',(-38.001,20.,-118.));
#19466=CARTESIAN_POINT('',(-6.,20.,-105.5));
#19467=CARTESIAN_POINT('Origin',(-6.,20.,-118.));
#19468=CARTESIAN_POINT('',(0.,20.,-105.5));
#19469=CARTESIAN_POINT('',(-38.001,20.,-105.5));
#19470=CARTESIAN_POINT('Origin',(0.,20.,-118.));
#19471=CARTESIAN_POINT('Origin',(-38.001,20.,-83.));
#19472=CARTESIAN_POINT('',(-6.,20.,-70.5));
#19473=CARTESIAN_POINT('Origin',(-6.,20.,-83.));
#19474=CARTESIAN_POINT('',(0.,20.,-70.5));
#19475=CARTESIAN_POINT('',(-38.001,20.,-70.5));
#19476=CARTESIAN_POINT('Origin',(0.,20.,-83.));
#19477=CARTESIAN_POINT('Origin',(12.,-6.93889390390723E-15,3.46944695195361E-15));
#19478=CARTESIAN_POINT('',(1.31131748603704,10.,5.45454545454546));
#19479=CARTESIAN_POINT('',(12.,10.,-12.));
#19480=CARTESIAN_POINT('Origin',(12.,10.,3.46944695195361E-15));
#19481=CARTESIAN_POINT('',(12.,30.,-12.));
#19482=CARTESIAN_POINT('',(12.,-0.00100000000000794,-12.));
#19483=CARTESIAN_POINT('',(1.31131748603704,30.,5.45454545454546));
#19484=CARTESIAN_POINT('Origin',(12.,30.,3.46944695195361E-15));
#19485=CARTESIAN_POINT('',(1.31131748603704,-6.93889390390723E-15,5.45454545454546));
#19486=CARTESIAN_POINT('Origin',(12.,-6.93889390390723E-15,3.46944695195361E-15));
#19487=CARTESIAN_POINT('',(12.,10.,-8.));
#19488=CARTESIAN_POINT('Origin',(12.,10.,3.46944695195361E-15));
#19489=CARTESIAN_POINT('',(12.,30.,-8.));
#19490=CARTESIAN_POINT('',(12.,-6.93889390390723E-15,-8.));
#19491=CARTESIAN_POINT('Origin',(12.,30.,3.46944695195361E-15));
#19492=CARTESIAN_POINT('Origin',(-26.,40.,-12.));
#19493=CARTESIAN_POINT('',(-26.,30.,-4.));
#19494=CARTESIAN_POINT('Origin',(-26.,30.,-12.));
#19495=CARTESIAN_POINT('',(-26.,10.,-4.));
#19496=CARTESIAN_POINT('',(-26.,40.,-4.));
#19497=CARTESIAN_POINT('Origin',(-26.,10.,-12.));
#19498=CARTESIAN_POINT('Origin',(0.,40.,0.));
#19499=CARTESIAN_POINT('',(0.,30.,1.73472347597681E-15));
#19500=CARTESIAN_POINT('',(0.,30.,-22.));
#19501=CARTESIAN_POINT('',(-1.24683249835833E-15,30.,12.001));
#19502=CARTESIAN_POINT('',(4.87890977618477E-16,10.,-22.));
#19503=CARTESIAN_POINT('',(0.,10.,-22.));
#19504=CARTESIAN_POINT('',(3.46944695195361E-15,10.,1.73472347597681E-15));
#19505=CARTESIAN_POINT('',(4.87890977618477E-16,10.,12.001));
#19506=CARTESIAN_POINT('',(0.,0.,-10.));
#19507=CARTESIAN_POINT('',(0.,-1.22464679914735E-15,-10.));
#19508=CARTESIAN_POINT('',(0.,-6.93889390390723E-15,-134.));
#19509=CARTESIAN_POINT('',(0.,0.,0.));
#19510=CARTESIAN_POINT('',(0.,10.,-144.));
#19511=CARTESIAN_POINT('',(0.,10.,-144.));
#19512=CARTESIAN_POINT('',(0.,30.,-144.));
#19513=CARTESIAN_POINT('',(0.,40.,-144.));
#19514=CARTESIAN_POINT('',(0.,40.,-134.));
#19515=CARTESIAN_POINT('',(0.,40.,-134.));
#19516=CARTESIAN_POINT('',(0.,40.,-10.));
#19517=CARTESIAN_POINT('',(0.,40.,0.));
#19518=CARTESIAN_POINT('',(0.,30.,1.73472347597681E-15));
#19519=CARTESIAN_POINT('Origin',(-26.,40.,-12.));
#19520=CARTESIAN_POINT('',(-6.,40.,-10.));
#19521=CARTESIAN_POINT('',(24.001,40.,-10.));
#19522=CARTESIAN_POINT('',(-6.,40.,-134.));
#19523=CARTESIAN_POINT('',(-6.,40.,-134.));
#19524=CARTESIAN_POINT('',(-6.,40.,-24.));
#19525=CARTESIAN_POINT('Origin',(-26.,0.,-12.));
#19526=CARTESIAN_POINT('',(-6.,-1.22464679914735E-15,-10.));
#19527=CARTESIAN_POINT('',(24.001,-1.22464679914735E-15,-10.));
#19528=CARTESIAN_POINT('',(-6.,0.,-134.));
#19529=CARTESIAN_POINT('',(-6.,0.,-24.));
#19530=CARTESIAN_POINT('',(-26.,0.,-134.));
#19531=CARTESIAN_POINT('Origin',(0.,40.,0.));
#19532=CARTESIAN_POINT('',(-7.59591794226543,10.,2.37360262678768E-15));
#19533=CARTESIAN_POINT('',(-26.,10.,8.67361737988404E-15));
#19534=CARTESIAN_POINT('',(-6.,10.,1.73472347597681E-15));
#19535=CARTESIAN_POINT('',(-7.59591794226543,30.,3.27314145353471E-15));
#19536=CARTESIAN_POINT('',(-7.59591794226543,40.,3.04080396370184E-15));
#19537=CARTESIAN_POINT('',(-26.,30.,8.67361737988404E-15));
#19538=CARTESIAN_POINT('',(-6.,30.,1.73472347597681E-15));
#19539=CARTESIAN_POINT('',(-26.,40.,8.67361737988404E-15));
#19540=CARTESIAN_POINT('Origin',(0.,40.,-144.));
#19541=CARTESIAN_POINT('',(-6.,10.,-144.));
#19542=CARTESIAN_POINT('',(0.,10.,-144.));
#19543=CARTESIAN_POINT('',(-6.,30.,-144.));
#19544=CARTESIAN_POINT('',(-6.,40.,-144.));
#19545=CARTESIAN_POINT('',(0.,30.,-144.));
#19546=CARTESIAN_POINT('Origin',(-6.,40.,-24.));
#19547=CARTESIAN_POINT('',(-6.,10.,1.73472347597681E-15));
#19548=CARTESIAN_POINT('',(-6.,-1.22464679914735E-15,-10.));
#19549=CARTESIAN_POINT('',(-6.,10.,-34.));
#19550=CARTESIAN_POINT('',(-6.,10.,12.001));
#19551=CARTESIAN_POINT('',(-6.,30.,-34.));
#19552=CARTESIAN_POINT('',(-6.,30.,-34.));
#19553=CARTESIAN_POINT('',(-6.,30.,2.77555756156289E-15));
#19554=CARTESIAN_POINT('',(-6.,30.,12.001));
#19555=CARTESIAN_POINT('',(-6.,30.,1.73472347597681E-15));
#19556=CARTESIAN_POINT('',(-6.,40.,-134.));
#19557=CARTESIAN_POINT('',(-6.,10.,-144.));
#19558=CARTESIAN_POINT('Origin',(-6.,40.,-24.));
#19559=CARTESIAN_POINT('',(-16.,30.,-24.));
#19560=CARTESIAN_POINT('',(-26.,30.,-24.));
#19561=CARTESIAN_POINT('',(-6.,30.,-24.));
#19562=CARTESIAN_POINT('',(-16.,10.,-24.));
#19563=CARTESIAN_POINT('',(-16.,10.,-24.));
#19564=CARTESIAN_POINT('',(-26.,10.,-24.));
#19565=CARTESIAN_POINT('',(-6.,10.,-24.));
#19566=CARTESIAN_POINT('',(-26.,40.,-24.));
#19567=CARTESIAN_POINT('Origin',(-26.,40.,-12.));
#19568=CARTESIAN_POINT('Origin',(-26.,10.,-12.));
#19569=CARTESIAN_POINT('Origin',(-26.,30.,-12.));
#19570=CARTESIAN_POINT('Origin',(0.,10.,-144.));
#19571=CARTESIAN_POINT('Origin',(-26.,40.,-134.));
#19572=CARTESIAN_POINT('Origin',(-6.,30.,12.001));
#19573=CARTESIAN_POINT('Origin',(-7.59591794226543,30.,10.));
#19574=CARTESIAN_POINT('',(10.,30.,-12.));
#19575=CARTESIAN_POINT('',(12.,30.,-12.));
#19576=CARTESIAN_POINT('Origin',(10.,30.,-22.));
#19577=CARTESIAN_POINT('',(24.001,30.,-2.42878633871514E-15));
#19578=CARTESIAN_POINT('Origin',(-16.,30.,-34.));
#19579=CARTESIAN_POINT('Origin',(4.87890977618477E-16,10.,12.001));
#19580=CARTESIAN_POINT('',(10.,10.,-12.));
#19581=CARTESIAN_POINT('',(12.,10.,-12.));
#19582=CARTESIAN_POINT('Origin',(-7.59591794226543,10.,10.));
#19583=CARTESIAN_POINT('Origin',(-16.,10.,-34.));
#19584=CARTESIAN_POINT('',(-3.67579230942105E-15,10.,8.67361737988404E-15));
#19585=CARTESIAN_POINT('Origin',(10.,10.,-22.));
#19586=CARTESIAN_POINT('Origin',(-16.,40.,-34.));
#19587=CARTESIAN_POINT('Origin',(24.001,30.,1.73472347597681E-15));
#19588=CARTESIAN_POINT('Origin',(24.001,-1.22464679914735E-15,-10.));
#19589=CARTESIAN_POINT('Origin',(12.,-0.00100000000000794,-12.));
#19590=CARTESIAN_POINT('',(10.,30.,-12.));
#19591=CARTESIAN_POINT('Origin',(10.,-0.00100000000000794,-22.));
#19592=CARTESIAN_POINT('Origin',(-7.59591794226543,-6.93889390390723E-15,
10.));
#20151=UNCERTAINTY_MEASURE_WITH_UNIT(LENGTH_MEASURE(0.01),#20177,
'DISTANCE_ACCURACY_VALUE',
'Maximum model space distance between geometric entities at asserted c
onnectivities');
#20160=UNCERTAINTY_MEASURE_WITH_UNIT(LENGTH_MEASURE(0.01),#20177,
'DISTANCE_ACCURACY_VALUE',
'Maximum model space distance between geometric entities at asserted c
onnectivities');
#20167=(
GEOMETRIC_REPRESENTATION_CONTEXT(3)
GLOBAL_UNCERTAINTY_ASSIGNED_CONTEXT((#20151))
GLOBAL_UNIT_ASSIGNED_CONTEXT((#20177,#20179,#20180))
REPRESENTATION_CONTEXT('','3D')
);
#20176=(
GEOMETRIC_REPRESENTATION_CONTEXT(3)
GLOBAL_UNCERTAINTY_ASSIGNED_CONTEXT((#20160))
GLOBAL_UNIT_ASSIGNED_CONTEXT((#20177,#20179,#20180))
REPRESENTATION_CONTEXT('','3D')
);
#20177=(
LENGTH_UNIT()
NAMED_UNIT(*)
SI_UNIT(.MILLI.,.METRE.)
);
#20179=(
NAMED_UNIT(*)
PLANE_ANGLE_UNIT()
SI_UNIT($,.RADIAN.)
);
#20180=(
NAMED_UNIT(*)
SI_UNIT($,.STERADIAN.)
SOLID_ANGLE_UNIT()
);
#20187=SHAPE_DEFINITION_REPRESENTATION(#20202,#20261);
#20202=PRODUCT_DEFINITION_SHAPE('',$,#20277);
#20261=SHAPE_REPRESENTATION('',(#11911),#20167);
#20270=PRODUCT_DEFINITION_CONTEXT('part definition',#20317,'design');
#20277=PRODUCT_DEFINITION('Gripper Finger','Gripper Finger',#20292,#20270);
#20292=PRODUCT_DEFINITION_FORMATION('',$,#20325);
#20317=APPLICATION_CONTEXT(
'Core Data for Automotive Mechanical Design Process');
#20318=PRODUCT_CONTEXT('part definition',#20317,'mechanical');
#20325=PRODUCT('Gripper Finger','Gripper Finger',$,(#20318));
#20337=PRESENTATION_STYLE_ASSIGNMENT((#20342));
#20342=SURFACE_STYLE_USAGE(.BOTH.,#20347);
#20347=SURFACE_SIDE_STYLE('',(#20352));
#20352=SURFACE_STYLE_FILL_AREA(#20357);
#20357=FILL_AREA_STYLE('Opaque(31,36,43)',(#20362));
#20362=FILL_AREA_STYLE_COLOUR('Opaque(31,36,43)',#20367);
#20367=COLOUR_RGB('Opaque(31,36,43)',0.12156862745098,0.141176470588235,
0.168627450980392);
ENDSEC;
END-ISO-10303-21;
